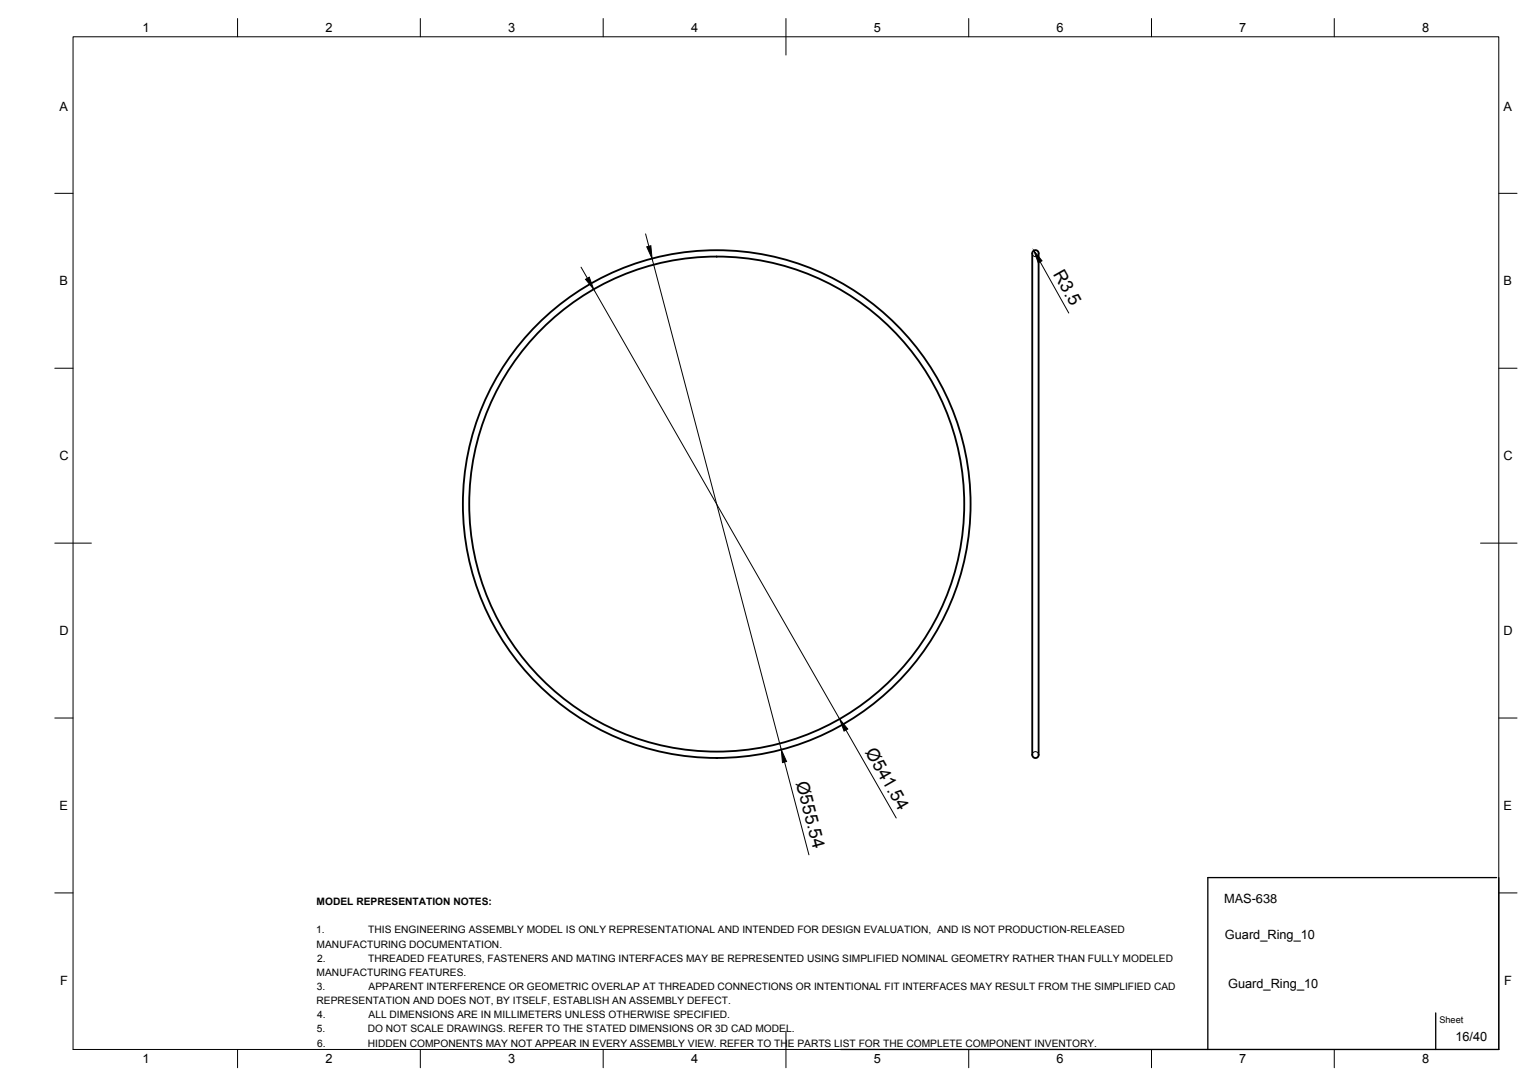
ISO-10303-21;
HEADER;
FILE_DESCRIPTION((''),'2;1');
FILE_NAME('Guard_Ring_10.step','2026-10-09T12:00:21-07:00',(''),(''),'','','');
FILE_SCHEMA (('AUTOMOTIVE_DESIGN { 1 0 10303 214 3 1 1 }'));
ENDSEC;
DATA;
#10=MECHANICAL_DESIGN_GEOMETRIC_PRESENTATION_REPRESENTATION('',(#409,#410),#10334);
#343=SHAPE_REPRESENTATION_RELATIONSHIP('SRR','None',#10459,#375) ;
#375=ADVANCED_BREP_SHAPE_REPRESENTATION('',(#447),#10311) ;
#409=STYLED_ITEM('',(#10631),#3376) ;
#410=STYLED_ITEM('',(#10632),#447) ;
#447=MANIFOLD_SOLID_BREP('Body1',#3569) ;
#868=FACE_OUTER_BOUND('',#1068,.T.) ;
#1068=EDGE_LOOP('',(#2385,#2386,#2387,#2388)) ;
#1294=CIRCLE('',#4011,0.349999999999999) ;
#1295=CIRCLE('',#4012,27.0768144613668) ;
#1522=VERTEX_POINT('',#5698) ;
#1849=EDGE_CURVE('',#1522,#1522,#1294,.T.) ;
#1850=EDGE_CURVE('',#1522,#1522,#1295,.T.) ;
#2385=ORIENTED_EDGE('',*,*,#1849,.F.) ;
#2386=ORIENTED_EDGE('',*,*,#1850,.T.) ;
#2387=ORIENTED_EDGE('',*,*,#1849,.T.) ;
#2388=ORIENTED_EDGE('',*,*,#1850,.F.) ;
#3314=TOROIDAL_SURFACE('',#4010,27.4268144613668,0.349999999999999) ;
#3376=ADVANCED_FACE('',(#868),#3314,.T.) ;
#3569=CLOSED_SHELL('',(#3376)) ;
#4009=AXIS2_PLACEMENT_3D('',#5696,#4579,#4580) ;
#4010=AXIS2_PLACEMENT_3D('',#5697,#4581,#4582) ;
#4011=AXIS2_PLACEMENT_3D('',#5699,#4583,#4584) ;
#4012=AXIS2_PLACEMENT_3D('',#5700,#4585,#4586) ;
#4579=DIRECTION('axis',(0.,0.,1.)) ;
#4580=DIRECTION('refdir',(1.,0.,0.)) ;
#4581=DIRECTION('center_axis',(-6.42891162084177E-17,-1.,-1.01883556321148E-16)) ;
#4582=DIRECTION('ref_axis',(1.,0.,0.)) ;
#4583=DIRECTION('center_axis',(0.,1.01883556321148E-16,-1.)) ;
#4584=DIRECTION('ref_axis',(-1.,0.,0.)) ;
#4585=DIRECTION('center_axis',(6.42891162084177E-17,1.,1.01883556321148E-16)) ;
#4586=DIRECTION('ref_axis',(1.,-6.42891162084177E-17,-6.55000379205715E-33)) ;
#5696=CARTESIAN_POINT('',(0.,0.,0.)) ;
#5697=CARTESIAN_POINT('Origin',(23.47768801576,67.3831179463143,68.2224337400009)) ;
#5698=CARTESIAN_POINT('',(-3.5991264456068,67.3831179463143,68.2224337400009)) ;
#5699=CARTESIAN_POINT('Origin',(-3.9491264456068,67.3831179463143,68.2224337400009)) ;
#5700=CARTESIAN_POINT('Origin',(23.47768801576,67.3831179463143,68.2224337400009)) ;
#10274=UNCERTAINTY_MEASURE_WITH_UNIT(LENGTH_MEASURE(0.001),#10335,
'DISTANCE_ACCURACY_VALUE',
'Maximum model space distance between geometric entities at asserted c
onnectivities') ;
#10297=UNCERTAINTY_MEASURE_WITH_UNIT(LENGTH_MEASURE(0.001),#10335,
'DISTANCE_ACCURACY_VALUE',
'Maximum model space distance between geometric entities at asserted c
onnectivities') ;
#10311=(
GEOMETRIC_REPRESENTATION_CONTEXT(3)
GLOBAL_UNCERTAINTY_ASSIGNED_CONTEXT((#10274))
GLOBAL_UNIT_ASSIGNED_CONTEXT((#10335,#10337,#10338))
REPRESENTATION_CONTEXT('','3D')
) ;
#10334=(
GEOMETRIC_REPRESENTATION_CONTEXT(3)
GLOBAL_UNCERTAINTY_ASSIGNED_CONTEXT((#10297))
GLOBAL_UNIT_ASSIGNED_CONTEXT((#10335,#10337,#10338))
REPRESENTATION_CONTEXT('','3D')
) ;
#10335=(
LENGTH_UNIT()
NAMED_UNIT(*)
SI_UNIT(.CENTI.,.METRE.)
) ;
#10337=(
NAMED_UNIT(*)
PLANE_ANGLE_UNIT()
SI_UNIT($,.RADIAN.)
) ;
#10338=(
NAMED_UNIT(*)
SI_UNIT($,.STERADIAN.)
SOLID_ANGLE_UNIT()
) ;
#10352=SHAPE_DEFINITION_REPRESENTATION(#10388,#10459) ;
#10388=PRODUCT_DEFINITION_SHAPE('',$,#10496) ;
#10459=SHAPE_REPRESENTATION('',(#4009),#10311) ;
#10482=PRODUCT_DEFINITION_CONTEXT('part definition',#10592,'design') ;
#10496=PRODUCT_DEFINITION('Guard_Ring_10','Guard_Ring_10',#10532,#10482) ;
#10532=PRODUCT_DEFINITION_FORMATION('',$,#10607) ;
#10592=APPLICATION_CONTEXT(
'Core Data for Automotive Mechanical Design Process') ;
#10593=PRODUCT_CONTEXT('part definition',#10592,'mechanical') ;
#10607=PRODUCT('Guard_Ring_10','Guard_Ring_10',$,(#10593)) ;
#10631=PRESENTATION_STYLE_ASSIGNMENT((#10635)) ;
#10632=PRESENTATION_STYLE_ASSIGNMENT((#10636)) ;
#10635=SURFACE_STYLE_USAGE(.BOTH.,#10639) ;
#10636=SURFACE_STYLE_USAGE(.BOTH.,#10640) ;
#10639=SURFACE_SIDE_STYLE('',(#10643)) ;
#10640=SURFACE_SIDE_STYLE('',(#10644)) ;
#10643=SURFACE_STYLE_FILL_AREA(#10647) ;
#10644=SURFACE_STYLE_FILL_AREA(#10648) ;
#10647=FILL_AREA_STYLE('Opaque(25,25,25)',(#10651)) ;
#10648=FILL_AREA_STYLE('Opaque(202,209,238)',(#10652)) ;
#10651=FILL_AREA_STYLE_COLOUR('Opaque(25,25,25)',#10655) ;
#10652=FILL_AREA_STYLE_COLOUR('Opaque(202,209,238)',#10656) ;
#10655=COLOUR_RGB('Opaque(25,25,25)', 0.09019608, 0.27058824, 0.51372549) ;
#10656=COLOUR_RGB('Opaque(202,209,238)', 0.40784314, 0.44705882, 0.49803922) ;
ENDSEC;
END-ISO-10303-21;
